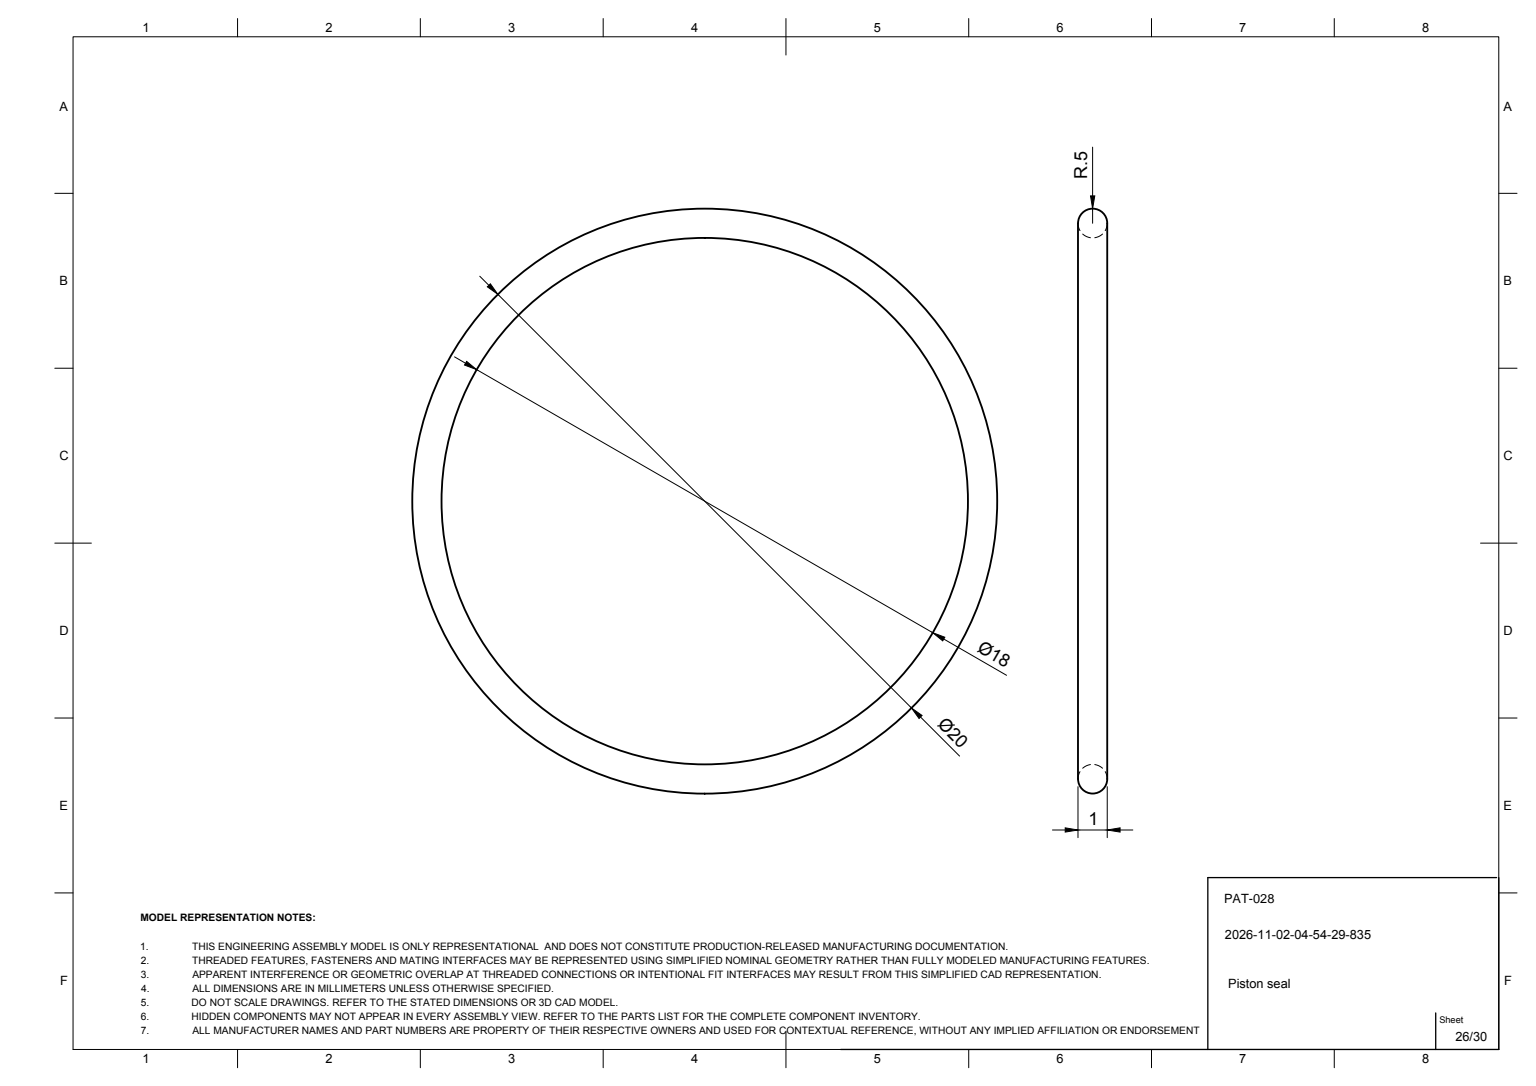
ISO-10303-21;
HEADER;
/* Generated by software containing ST-Developer
 * from STEP Tools, Inc. (www.steptools.com) 
 */

FILE_DESCRIPTION(
/* description */ ('Cylinder foot and clevis mount kit'),
/* implementation_level */ '2;1');

FILE_NAME(
/* name */ 'Piston seal.step',
/* time_stamp */ '2026-10-27T20:10:43-07:00',
/* author */ (''),
/* organization */ (''),
/* preprocessor_version */ 'ST-DEVELOPER v20.2',
/* originating_system */ 'Autodesk Translation Framework v15.17.0.0',
/* authorisation */ '');

FILE_SCHEMA (('AUTOMOTIVE_DESIGN { 1 0 10303 214 3 1 1 }'));
ENDSEC;

DATA;
#10=MECHANICAL_DESIGN_GEOMETRIC_PRESENTATION_REPRESENTATION('',(#358),#9102);
#33=TOROIDAL_SURFACE('',#5760,0.95,0.05);
#302=SHAPE_REPRESENTATION_RELATIONSHIP('SRR','None',#9251,#330);
#330=ADVANCED_BREP_SHAPE_REPRESENTATION('',(#385),#9094);
#358=STYLED_ITEM('',(#9467),#385);
#385=MANIFOLD_SOLID_BREP('Body1',#4945);
#933=FACE_OUTER_BOUND('',#1326,.T.);
#1326=EDGE_LOOP('',(#4239,#4240,#4241,#4242));
#2285=CIRCLE('',#5761,0.05);
#2286=CIRCLE('',#5762,0.9);
#2621=VERTEX_POINT('',#8582);
#3174=EDGE_CURVE('',#2621,#2621,#2285,.T.);
#3175=EDGE_CURVE('',#2621,#2621,#2286,.T.);
#4239=ORIENTED_EDGE('',*,*,#3174,.F.);
#4240=ORIENTED_EDGE('',*,*,#3175,.T.);
#4241=ORIENTED_EDGE('',*,*,#3174,.T.);
#4242=ORIENTED_EDGE('',*,*,#3175,.F.);
#4856=ADVANCED_FACE('',(#933),#33,.T.);
#4945=CLOSED_SHELL('',(#4856));
#5759=AXIS2_PLACEMENT_3D('',#8580,#7142,#7143);
#5760=AXIS2_PLACEMENT_3D('',#8581,#7144,#7145);
#5761=AXIS2_PLACEMENT_3D('',#8583,#7146,#7147);
#5762=AXIS2_PLACEMENT_3D('',#8584,#7148,#7149);
#7142=DIRECTION('axis',(0.,0.,1.));
#7143=DIRECTION('refdir',(1.,0.,0.));
#7144=DIRECTION('center_axis',(0.,-1.,0.));
#7145=DIRECTION('ref_axis',(0.,0.,-1.));
#7146=DIRECTION('center_axis',(-1.,0.,-1.22464679914735E-16));
#7147=DIRECTION('ref_axis',(-1.22464679914735E-16,0.,1.));
#7148=DIRECTION('center_axis',(0.,1.,0.));
#7149=DIRECTION('ref_axis',(0.,0.,-1.));
#8580=CARTESIAN_POINT('',(0.,0.,0.));
#8581=CARTESIAN_POINT('Origin',(0.,2.95,4.5));
#8582=CARTESIAN_POINT('',(-1.10218211923262E-16,2.95,5.4));
#8583=CARTESIAN_POINT('Origin',(-1.16341445918999E-16,2.95,5.45));
#8584=CARTESIAN_POINT('Origin',(0.,2.95,4.5));
#9061=UNCERTAINTY_MEASURE_WITH_UNIT(LENGTH_MEASURE(0.001),#9103,
'DISTANCE_ACCURACY_VALUE',
'Maximum model space distance between geometric entities at asserted c
onnectivities');
#9069=UNCERTAINTY_MEASURE_WITH_UNIT(LENGTH_MEASURE(0.001),#9103,
'DISTANCE_ACCURACY_VALUE',
'Maximum model space distance between geometric entities at asserted c
onnectivities');
#9094=(
GEOMETRIC_REPRESENTATION_CONTEXT(3)
GLOBAL_UNCERTAINTY_ASSIGNED_CONTEXT((#9061))
GLOBAL_UNIT_ASSIGNED_CONTEXT((#9103,#9105,#9106))
REPRESENTATION_CONTEXT('','3D')
);
#9102=(
GEOMETRIC_REPRESENTATION_CONTEXT(3)
GLOBAL_UNCERTAINTY_ASSIGNED_CONTEXT((#9069))
GLOBAL_UNIT_ASSIGNED_CONTEXT((#9103,#9105,#9106))
REPRESENTATION_CONTEXT('','3D')
);
#9103=(
LENGTH_UNIT()
NAMED_UNIT(*)
SI_UNIT(.CENTI.,.METRE.)
);
#9105=(
NAMED_UNIT(*)
PLANE_ANGLE_UNIT()
SI_UNIT($,.RADIAN.)
);
#9106=(
NAMED_UNIT(*)
SI_UNIT($,.STERADIAN.)
SOLID_ANGLE_UNIT()
);
#9131=SHAPE_DEFINITION_REPRESENTATION(#9206,#9251);
#9206=PRODUCT_DEFINITION_SHAPE('',$,#9284);
#9251=SHAPE_REPRESENTATION('',(#5759),#9094);
#9259=PRODUCT_DEFINITION_CONTEXT('part definition',#9357,'design');
#9284=PRODUCT_DEFINITION('Piston seal','Piston seal',#9316,#9259);
#9316=PRODUCT_DEFINITION_FORMATION('',$,#9383);
#9357=APPLICATION_CONTEXT(
'Core Data for Automotive Mechanical Design Process');
#9358=PRODUCT_CONTEXT('part definition',#9357,'mechanical');
#9383=PRODUCT('Piston seal','Piston seal','Piston seal',(#9358));
#9461=COLOUR_RGB('Black',0.12,0.14,0.17);
#9462=FILL_AREA_STYLE_COLOUR('',#9461);
#9463=FILL_AREA_STYLE('',(#9462));
#9464=SURFACE_STYLE_FILL_AREA(#9463);
#9465=SURFACE_SIDE_STYLE('',(#9464));
#9466=SURFACE_STYLE_USAGE(.BOTH.,#9465);
#9467=PRESENTATION_STYLE_ASSIGNMENT((#9466));
ENDSEC;
END-ISO-10303-21;
